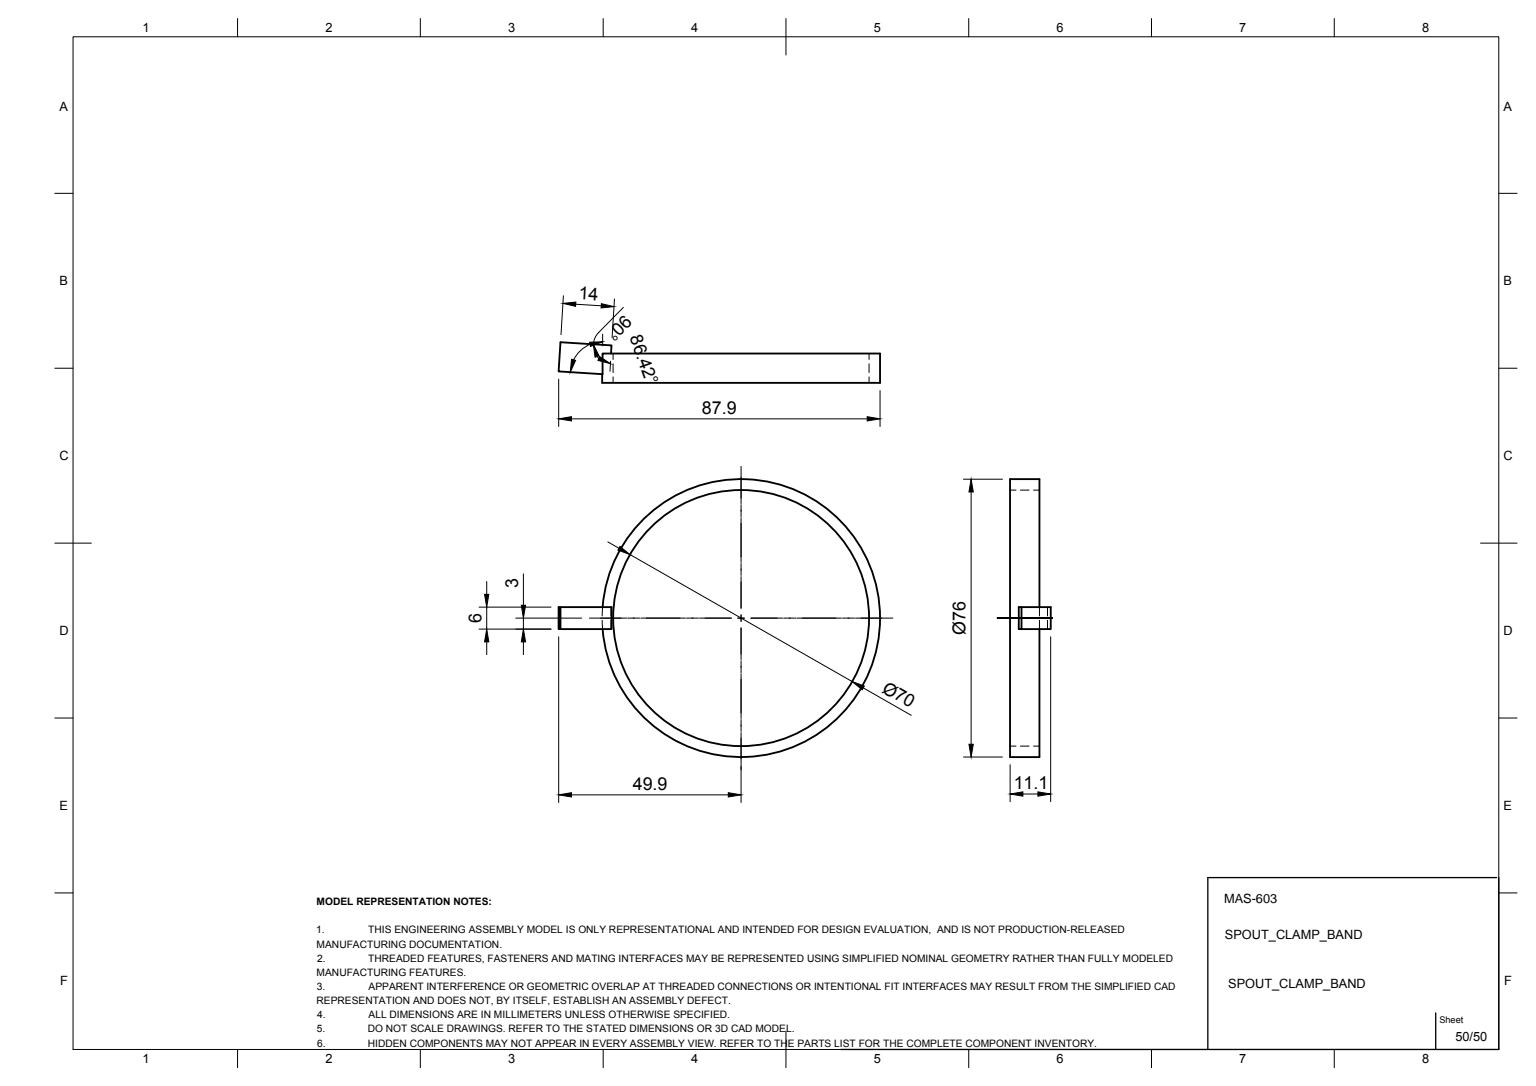
ISO-10303-21;
HEADER;
FILE_DESCRIPTION((''),'2;1');
FILE_NAME('SPOUT_CLAMP_BAND.step','2026-10-01T22:06:14-07:00',(''),(''),'','','');
FILE_SCHEMA (('AUTOMOTIVE_DESIGN { 1 0 10303 214 3 1 1 }'));
ENDSEC;
DATA;
#10=MECHANICAL_DESIGN_GEOMETRIC_PRESENTATION_REPRESENTATION('',(#1029),#50440);
#675=ELLIPSE('',#32186,3.80741464119683,3.8) ;
#928=SHAPE_REPRESENTATION_RELATIONSHIP('SRR','None',#50662,#973) ;
#973=ADVANCED_BREP_SHAPE_REPRESENTATION('',(#1082),#50431) ;
#1029=STYLED_ITEM('',(#50889),#1082) ;
#1082=MANIFOLD_SOLID_BREP('SPOUT_CLAMP_BAND',#28707) ;
#1398=FACE_BOUND('',#5656,.T.) ;
#1399=FACE_BOUND('',#5660,.T.) ;
#2289=PLANE('',#32184) ;
#2290=PLANE('',#32185) ;
#2291=PLANE('',#32187) ;
#2292=PLANE('',#32188) ;
#2293=PLANE('',#32189) ;
#2294=PLANE('',#32190) ;
#2295=PLANE('',#32191) ;
#2296=PLANE('',#32199) ;
#3809=FACE_OUTER_BOUND('',#5649,.T.) ;
#3810=FACE_OUTER_BOUND('',#5650,.T.) ;
#3811=FACE_OUTER_BOUND('',#5651,.T.) ;
#3812=FACE_OUTER_BOUND('',#5652,.T.) ;
#3813=FACE_OUTER_BOUND('',#5653,.T.) ;
#3814=FACE_OUTER_BOUND('',#5654,.T.) ;
#3815=FACE_OUTER_BOUND('',#5655,.T.) ;
#3816=FACE_OUTER_BOUND('',#5657,.T.) ;
#3817=FACE_OUTER_BOUND('',#5658,.T.) ;
#3818=FACE_OUTER_BOUND('',#5659,.T.) ;
#5649=EDGE_LOOP('',(#26259,#26260,#26261,#26262,#26263,#26264)) ;
#5650=EDGE_LOOP('',(#26265,#26266,#26267,#26268)) ;
#5651=EDGE_LOOP('',(#26269,#26270,#26271,#26272)) ;
#5652=EDGE_LOOP('',(#26273,#26274,#26275,#26276)) ;
#5653=EDGE_LOOP('',(#26277,#26278,#26279,#26280)) ;
#5654=EDGE_LOOP('',(#26281,#26282,#26283,#26284,#26285,#26286)) ;
#5655=EDGE_LOOP('',(#26287,#26288,#26289,#26290,#26291)) ;
#5656=EDGE_LOOP('',(#26292)) ;
#5657=EDGE_LOOP('',(#26293,#26294,#26295,#26296)) ;
#5658=EDGE_LOOP('',(#26297,#26298,#26299,#26300,#26301,#26302,#26303,#26304)) ;
#5659=EDGE_LOOP('',(#26305)) ;
#5660=EDGE_LOOP('',(#26306)) ;
#8105=LINE('',#49845,#10577) ;
#8106=LINE('',#49847,#10578) ;
#8107=LINE('',#49849,#10579) ;
#8108=LINE('',#49851,#10580) ;
#8109=LINE('',#49853,#10581) ;
#8110=LINE('',#49854,#10582) ;
#8111=LINE('',#49859,#10583) ;
#8112=LINE('',#49860,#10584) ;
#8113=LINE('',#49863,#10585) ;
#8114=LINE('',#49864,#10586) ;
#8115=LINE('',#49867,#10587) ;
#8116=LINE('',#49869,#10588) ;
#8117=LINE('',#49870,#10589) ;
#8118=LINE('',#49872,#10590) ;
#8119=LINE('',#49875,#10591) ;
#8120=LINE('',#49876,#10592) ;
#8121=LINE('',#49885,#10593) ;
#8122=LINE('',#49890,#10594) ;
#10577=VECTOR('',#40700,1.) ;
#10578=VECTOR('',#40701,1.) ;
#10579=VECTOR('',#40702,1.) ;
#10580=VECTOR('',#40703,1.) ;
#10581=VECTOR('',#40704,1.) ;
#10582=VECTOR('',#40705,1.) ;
#10583=VECTOR('',#40710,1.) ;
#10584=VECTOR('',#40711,1.) ;
#10585=VECTOR('',#40714,1.) ;
#10586=VECTOR('',#40715,1.) ;
#10587=VECTOR('',#40718,1.) ;
#10588=VECTOR('',#40719,1.) ;
#10589=VECTOR('',#40720,1.) ;
#10590=VECTOR('',#40723,1.) ;
#10591=VECTOR('',#40726,1.) ;
#10592=VECTOR('',#40727,1.) ;
#10593=VECTOR('',#40738,3.5) ;
#10594=VECTOR('',#40745,3.8) ;
#11797=CIRCLE('',#32192,3.8) ;
#11798=CIRCLE('',#32193,3.8) ;
#11799=CIRCLE('',#32194,3.5) ;
#11800=CIRCLE('',#32196,3.5) ;
#11801=CIRCLE('',#32198,3.8) ;
#14432=VERTEX_POINT('',#49843) ;
#14433=VERTEX_POINT('',#49844) ;
#14434=VERTEX_POINT('',#49846) ;
#14435=VERTEX_POINT('',#49848) ;
#14436=VERTEX_POINT('',#49850) ;
#14437=VERTEX_POINT('',#49852) ;
#14438=VERTEX_POINT('',#49856) ;
#14439=VERTEX_POINT('',#49858) ;
#14440=VERTEX_POINT('',#49862) ;
#14441=VERTEX_POINT('',#49866) ;
#14442=VERTEX_POINT('',#49868) ;
#14443=VERTEX_POINT('',#49874) ;
#14444=VERTEX_POINT('',#49878) ;
#14445=VERTEX_POINT('',#49881) ;
#14446=VERTEX_POINT('',#49884) ;
#14447=VERTEX_POINT('',#49888) ;
#18395=EDGE_CURVE('',#14432,#14433,#8105,.T.) ;
#18396=EDGE_CURVE('',#14434,#14432,#8106,.T.) ;
#18397=EDGE_CURVE('',#14435,#14434,#8107,.T.) ;
#18398=EDGE_CURVE('',#14436,#14435,#8108,.T.) ;
#18399=EDGE_CURVE('',#14436,#14437,#8109,.T.) ;
#18400=EDGE_CURVE('',#14433,#14437,#8110,.T.) ;
#18401=EDGE_CURVE('',#14438,#14434,#675,.T.) ;
#18402=EDGE_CURVE('',#14439,#14438,#8111,.T.) ;
#18403=EDGE_CURVE('',#14435,#14439,#8112,.T.) ;
#18404=EDGE_CURVE('',#14439,#14440,#8113,.T.) ;
#18405=EDGE_CURVE('',#14440,#14436,#8114,.T.) ;
#18406=EDGE_CURVE('',#14433,#14441,#8115,.T.) ;
#18407=EDGE_CURVE('',#14437,#14442,#8116,.T.) ;
#18408=EDGE_CURVE('',#14442,#14441,#8117,.T.) ;
#18409=EDGE_CURVE('',#14440,#14442,#8118,.T.) ;
#18410=EDGE_CURVE('',#14441,#14443,#8119,.T.) ;
#18411=EDGE_CURVE('',#14443,#14438,#8120,.T.) ;
#18412=EDGE_CURVE('',#14443,#14444,#11797,.T.) ;
#18413=EDGE_CURVE('',#14444,#14432,#11798,.T.) ;
#18414=EDGE_CURVE('',#14445,#14445,#11799,.T.) ;
#18415=EDGE_CURVE('',#14445,#14446,#8121,.T.) ;
#18416=EDGE_CURVE('',#14446,#14446,#11800,.T.) ;
#18417=EDGE_CURVE('',#14447,#14447,#11801,.T.) ;
#18418=EDGE_CURVE('',#14447,#14444,#8122,.T.) ;
#26259=ORIENTED_EDGE('',*,*,#18395,.F.) ;
#26260=ORIENTED_EDGE('',*,*,#18396,.F.) ;
#26261=ORIENTED_EDGE('',*,*,#18397,.F.) ;
#26262=ORIENTED_EDGE('',*,*,#18398,.F.) ;
#26263=ORIENTED_EDGE('',*,*,#18399,.T.) ;
#26264=ORIENTED_EDGE('',*,*,#18400,.F.) ;
#26265=ORIENTED_EDGE('',*,*,#18401,.F.) ;
#26266=ORIENTED_EDGE('',*,*,#18402,.F.) ;
#26267=ORIENTED_EDGE('',*,*,#18403,.F.) ;
#26268=ORIENTED_EDGE('',*,*,#18397,.T.) ;
#26269=ORIENTED_EDGE('',*,*,#18403,.T.) ;
#26270=ORIENTED_EDGE('',*,*,#18404,.T.) ;
#26271=ORIENTED_EDGE('',*,*,#18405,.T.) ;
#26272=ORIENTED_EDGE('',*,*,#18398,.T.) ;
#26273=ORIENTED_EDGE('',*,*,#18406,.F.) ;
#26274=ORIENTED_EDGE('',*,*,#18400,.T.) ;
#26275=ORIENTED_EDGE('',*,*,#18407,.T.) ;
#26276=ORIENTED_EDGE('',*,*,#18408,.T.) ;
#26277=ORIENTED_EDGE('',*,*,#18409,.T.) ;
#26278=ORIENTED_EDGE('',*,*,#18407,.F.) ;
#26279=ORIENTED_EDGE('',*,*,#18399,.F.) ;
#26280=ORIENTED_EDGE('',*,*,#18405,.F.) ;
#26281=ORIENTED_EDGE('',*,*,#18410,.F.) ;
#26282=ORIENTED_EDGE('',*,*,#18408,.F.) ;
#26283=ORIENTED_EDGE('',*,*,#18409,.F.) ;
#26284=ORIENTED_EDGE('',*,*,#18404,.F.) ;
#26285=ORIENTED_EDGE('',*,*,#18402,.T.) ;
#26286=ORIENTED_EDGE('',*,*,#18411,.F.) ;
#26287=ORIENTED_EDGE('',*,*,#18395,.T.) ;
#26288=ORIENTED_EDGE('',*,*,#18406,.T.) ;
#26289=ORIENTED_EDGE('',*,*,#18410,.T.) ;
#26290=ORIENTED_EDGE('',*,*,#18412,.T.) ;
#26291=ORIENTED_EDGE('',*,*,#18413,.T.) ;
#26292=ORIENTED_EDGE('',*,*,#18414,.T.) ;
#26293=ORIENTED_EDGE('',*,*,#18414,.F.) ;
#26294=ORIENTED_EDGE('',*,*,#18415,.T.) ;
#26295=ORIENTED_EDGE('',*,*,#18416,.F.) ;
#26296=ORIENTED_EDGE('',*,*,#18415,.F.) ;
#26297=ORIENTED_EDGE('',*,*,#18417,.F.) ;
#26298=ORIENTED_EDGE('',*,*,#18418,.T.) ;
#26299=ORIENTED_EDGE('',*,*,#18412,.F.) ;
#26300=ORIENTED_EDGE('',*,*,#18411,.T.) ;
#26301=ORIENTED_EDGE('',*,*,#18401,.T.) ;
#26302=ORIENTED_EDGE('',*,*,#18396,.T.) ;
#26303=ORIENTED_EDGE('',*,*,#18413,.F.) ;
#26304=ORIENTED_EDGE('',*,*,#18418,.F.) ;
#26305=ORIENTED_EDGE('',*,*,#18417,.T.) ;
#26306=ORIENTED_EDGE('',*,*,#18416,.T.) ;
#27052=CYLINDRICAL_SURFACE('',#32195,3.5) ;
#27053=CYLINDRICAL_SURFACE('',#32197,3.8) ;
#28544=ADVANCED_FACE('',(#3809),#2289,.F.) ;
#28545=ADVANCED_FACE('',(#3810),#2290,.F.) ;
#28546=ADVANCED_FACE('',(#3811),#2291,.T.) ;
#28547=ADVANCED_FACE('',(#3812),#2292,.F.) ;
#28548=ADVANCED_FACE('',(#3813),#2293,.F.) ;
#28549=ADVANCED_FACE('',(#3814),#2294,.F.) ;
#28550=ADVANCED_FACE('',(#3815,#1398),#2295,.T.) ;
#28551=ADVANCED_FACE('',(#3816),#27052,.F.) ;
#28552=ADVANCED_FACE('',(#3817),#27053,.T.) ;
#28553=ADVANCED_FACE('',(#3818,#1399),#2296,.T.) ;
#28707=CLOSED_SHELL('',(#28544,#28545,#28546,#28547,#28548,#28549,#28550,
#28551,#28552,#28553)) ;
#32183=AXIS2_PLACEMENT_3D('',#49841,#40696,#40697) ;
#32184=AXIS2_PLACEMENT_3D('',#49842,#40698,#40699) ;
#32185=AXIS2_PLACEMENT_3D('',#49855,#40706,#40707) ;
#32186=AXIS2_PLACEMENT_3D('',#49857,#40708,#40709) ;
#32187=AXIS2_PLACEMENT_3D('',#49861,#40712,#40713) ;
#32188=AXIS2_PLACEMENT_3D('',#49865,#40716,#40717) ;
#32189=AXIS2_PLACEMENT_3D('',#49871,#40721,#40722) ;
#32190=AXIS2_PLACEMENT_3D('',#49873,#40724,#40725) ;
#32191=AXIS2_PLACEMENT_3D('',#49877,#40728,#40729) ;
#32192=AXIS2_PLACEMENT_3D('',#49879,#40730,#40731) ;
#32193=AXIS2_PLACEMENT_3D('',#49880,#40732,#40733) ;
#32194=AXIS2_PLACEMENT_3D('',#49882,#40734,#40735) ;
#32195=AXIS2_PLACEMENT_3D('',#49883,#40736,#40737) ;
#32196=AXIS2_PLACEMENT_3D('',#49886,#40739,#40740) ;
#32197=AXIS2_PLACEMENT_3D('',#49887,#40741,#40742) ;
#32198=AXIS2_PLACEMENT_3D('',#49889,#40743,#40744) ;
#32199=AXIS2_PLACEMENT_3D('',#49891,#40746,#40747) ;
#40696=DIRECTION('axis',(0.,0.,1.)) ;
#40697=DIRECTION('refdir',(1.,0.,0.)) ;
#40698=DIRECTION('center_axis',(0.,1.,0.)) ;
#40699=DIRECTION('ref_axis',(0.,0.,1.)) ;
#40700=DIRECTION('',(-0.0623782861551789,0.,-0.998052578482889)) ;
#40701=DIRECTION('',(-0.998052578482889,0.,0.0623782861551789)) ;
#40702=DIRECTION('',(0.,0.,-1.)) ;
#40703=DIRECTION('',(1.,0.,0.)) ;
#40704=DIRECTION('',(0.,0.,-1.)) ;
#40705=DIRECTION('',(-1.,0.,0.)) ;
#40706=DIRECTION('center_axis',(-1.,0.,0.)) ;
#40707=DIRECTION('ref_axis',(0.,0.,1.)) ;
#40708=DIRECTION('center_axis',(1.,0.,0.)) ;
#40709=DIRECTION('ref_axis',(0.,0.,1.)) ;
#40710=DIRECTION('',(0.,0.,-1.)) ;
#40711=DIRECTION('',(0.,1.,0.)) ;
#40712=DIRECTION('center_axis',(0.,0.,1.)) ;
#40713=DIRECTION('ref_axis',(1.,0.,0.)) ;
#40714=DIRECTION('',(-1.,0.,0.)) ;
#40715=DIRECTION('',(0.,-1.,0.)) ;
#40716=DIRECTION('center_axis',(0.,0.,1.)) ;
#40717=DIRECTION('ref_axis',(1.,0.,0.)) ;
#40718=DIRECTION('',(0.,1.,0.)) ;
#40719=DIRECTION('',(0.,1.,0.)) ;
#40720=DIRECTION('',(1.,0.,0.)) ;
#40721=DIRECTION('center_axis',(1.,0.,0.)) ;
#40722=DIRECTION('ref_axis',(0.,0.,-1.)) ;
#40723=DIRECTION('',(0.,0.,-1.)) ;
#40724=DIRECTION('center_axis',(0.,-1.,0.)) ;
#40725=DIRECTION('ref_axis',(0.,0.,-1.)) ;
#40726=DIRECTION('',(0.0623782861551789,0.,0.998052578482889)) ;
#40727=DIRECTION('',(0.998052578482889,0.,-0.0623782861551789)) ;
#40728=DIRECTION('center_axis',(-0.998052578482889,0.,0.0623782861551789)) ;
#40729=DIRECTION('ref_axis',(-0.0623782861551789,0.,-0.998052578482889)) ;
#40730=DIRECTION('center_axis',(-0.998052578482889,0.,0.0623782861551789)) ;
#40731=DIRECTION('ref_axis',(0.0623782861551789,0.,0.998052578482889)) ;
#40732=DIRECTION('center_axis',(-0.998052578482889,0.,0.0623782861551789)) ;
#40733=DIRECTION('ref_axis',(0.0623782861551789,0.,0.998052578482889)) ;
#40734=DIRECTION('center_axis',(0.998052578482889,0.,-0.0623782861551789)) ;
#40735=DIRECTION('ref_axis',(0.0623782861551792,0.,0.998052578482889)) ;
#40736=DIRECTION('center_axis',(0.998052578482889,0.,-0.0623782861551792)) ;
#40737=DIRECTION('ref_axis',(0.0623782861551792,0.,0.998052578482889)) ;
#40738=DIRECTION('',(0.998052578482889,0.,-0.0623782861551792)) ;
#40739=DIRECTION('center_axis',(-0.998052578482889,0.,0.0623782861551789)) ;
#40740=DIRECTION('ref_axis',(0.0623782861551792,0.,0.998052578482889)) ;
#40741=DIRECTION('center_axis',(0.998052578482889,0.,-0.0623782861551789)) ;
#40742=DIRECTION('ref_axis',(0.0623782861551789,0.,0.998052578482889)) ;
#40743=DIRECTION('center_axis',(0.998052578482889,0.,-0.0623782861551789)) ;
#40744=DIRECTION('ref_axis',(0.0623782861551789,0.,0.998052578482889)) ;
#40745=DIRECTION('',(-0.998052578482889,0.,0.0623782861551789)) ;
#40746=DIRECTION('center_axis',(0.998052578482889,0.,-0.0623782861551789)) ;
#40747=DIRECTION('ref_axis',(0.0623782861551789,0.,0.998052578482889)) ;
#49841=CARTESIAN_POINT('',(0.,0.,0.)) ;
#49842=CARTESIAN_POINT('Origin',(60.4,-0.3,15.5)) ;
#49843=CARTESIAN_POINT('',(60.2362976425517,-0.3,15.030762280827)) ;
#49844=CARTESIAN_POINT('',(60.221875,-0.3,14.8)) ;
#49845=CARTESIAN_POINT('',(60.1330739299611,-0.3,13.3791828793774)) ;
#49846=CARTESIAN_POINT('',(60.8,-0.3,14.9955308834865)) ;
#49847=CARTESIAN_POINT('',(60.6362976425517,-0.3,15.005762280827)) ;
#49848=CARTESIAN_POINT('',(60.8,-0.3,16.2)) ;
#49849=CARTESIAN_POINT('',(60.8,-0.3,15.5)) ;
#49850=CARTESIAN_POINT('',(60.,-0.3,16.2)) ;
#49851=CARTESIAN_POINT('',(60.4,-0.3,16.2)) ;
#49852=CARTESIAN_POINT('',(60.,-0.3,14.8)) ;
#49853=CARTESIAN_POINT('',(60.,-0.3,15.5)) ;
#49854=CARTESIAN_POINT('',(60.4,-0.3,14.8)) ;
#49855=CARTESIAN_POINT('Origin',(60.8,0.,15.5)) ;
#49856=CARTESIAN_POINT('',(60.8,0.3,14.9955308834865)) ;
#49857=CARTESIAN_POINT('Origin',(60.8,0.,11.2)) ;
#49858=CARTESIAN_POINT('',(60.8,0.3,16.2)) ;
#49859=CARTESIAN_POINT('',(60.8,0.3,15.5)) ;
#49860=CARTESIAN_POINT('',(60.8,0.,16.2)) ;
#49861=CARTESIAN_POINT('Origin',(60.4,0.,16.2)) ;
#49862=CARTESIAN_POINT('',(60.,0.3,16.2)) ;
#49863=CARTESIAN_POINT('',(60.4,0.3,16.2)) ;
#49864=CARTESIAN_POINT('',(60.,0.,16.2)) ;
#49865=CARTESIAN_POINT('Origin',(60.4,0.,14.8)) ;
#49866=CARTESIAN_POINT('',(60.221875,0.3,14.8)) ;
#49867=CARTESIAN_POINT('',(60.221875,0.,14.8)) ;
#49868=CARTESIAN_POINT('',(60.,0.3,14.8)) ;
#49869=CARTESIAN_POINT('',(60.,0.,14.8)) ;
#49870=CARTESIAN_POINT('',(60.4,0.3,14.8)) ;
#49871=CARTESIAN_POINT('Origin',(60.,0.,15.5)) ;
#49872=CARTESIAN_POINT('',(60.,0.3,15.5)) ;
#49873=CARTESIAN_POINT('Origin',(60.4,0.3,15.5)) ;
#49874=CARTESIAN_POINT('',(60.2362976425517,0.3,15.030762280827)) ;
#49875=CARTESIAN_POINT('',(60.1330739299611,0.3,13.3791828793774)) ;
#49876=CARTESIAN_POINT('',(60.6362976425517,0.3,15.005762280827)) ;
#49877=CARTESIAN_POINT('Origin',(60.,0.,11.25)) ;
#49878=CARTESIAN_POINT('',(59.7629625126103,4.65365783675994E-16,7.45740020176502)) ;
#49879=CARTESIAN_POINT('Origin',(60.,0.,11.25)) ;
#49880=CARTESIAN_POINT('Origin',(60.,0.,11.25)) ;
#49881=CARTESIAN_POINT('',(59.7816759984569,4.28626379701574E-16,7.75681597530989)) ;
#49882=CARTESIAN_POINT('Origin',(60.,0.,11.25)) ;
#49883=CARTESIAN_POINT('Origin',(60.4,0.,11.225)) ;
#49884=CARTESIAN_POINT('',(60.5816759984569,-4.28626379701574E-16,7.70681597530989)) ;
#49885=CARTESIAN_POINT('',(60.1816759984569,4.28626379701574E-16,7.73181597530989)) ;
#49886=CARTESIAN_POINT('Origin',(60.8,0.,11.2)) ;
#49887=CARTESIAN_POINT('Origin',(60.4,0.,11.225)) ;
#49888=CARTESIAN_POINT('',(60.5629625126103,4.65365783675994E-16,7.40740020176502)) ;
#49889=CARTESIAN_POINT('Origin',(60.8,0.,11.2)) ;
#49890=CARTESIAN_POINT('',(60.1629625126103,4.65365783675994E-16,7.43240020176502)) ;
#49891=CARTESIAN_POINT('Origin',(60.8,0.,11.2)) ;
#50378=UNCERTAINTY_MEASURE_WITH_UNIT(LENGTH_MEASURE(0.001),#50441,
'DISTANCE_ACCURACY_VALUE',
'Maximum model space distance between geometric entities at asserted c
onnectivities') ;
#50387=UNCERTAINTY_MEASURE_WITH_UNIT(LENGTH_MEASURE(0.001),#50441,
'DISTANCE_ACCURACY_VALUE',
'Maximum model space distance between geometric entities at asserted c
onnectivities') ;
#50431=(
GEOMETRIC_REPRESENTATION_CONTEXT(3)
GLOBAL_UNCERTAINTY_ASSIGNED_CONTEXT((#50378))
GLOBAL_UNIT_ASSIGNED_CONTEXT((#50441,#50443,#50444))
REPRESENTATION_CONTEXT('','3D')
) ;
#50440=(
GEOMETRIC_REPRESENTATION_CONTEXT(3)
GLOBAL_UNCERTAINTY_ASSIGNED_CONTEXT((#50387))
GLOBAL_UNIT_ASSIGNED_CONTEXT((#50441,#50443,#50444))
REPRESENTATION_CONTEXT('','3D')
) ;
#50441=(
LENGTH_UNIT()
NAMED_UNIT(*)
SI_UNIT(.CENTI.,.METRE.)
) ;
#50443=(
NAMED_UNIT(*)
PLANE_ANGLE_UNIT()
SI_UNIT($,.RADIAN.)
) ;
#50444=(
NAMED_UNIT(*)
SI_UNIT($,.STERADIAN.)
SOLID_ANGLE_UNIT()
) ;
#50488=SHAPE_DEFINITION_REPRESENTATION(#50578,#50662) ;
#50578=PRODUCT_DEFINITION_SHAPE('',$,#50715) ;
#50662=SHAPE_REPRESENTATION('',(#32183),#50431) ;
#50671=PRODUCT_DEFINITION_CONTEXT('part definition',#50829,'design') ;
#50715=PRODUCT_DEFINITION('SPOUT_CLAMP_BAND','SPOUT_CLAMP_BAND',
#50767,#50671) ;
#50767=PRODUCT_DEFINITION_FORMATION('',$,#50874) ;
#50829=APPLICATION_CONTEXT(
'Core Data for Automotive Mechanical Design Process') ;
#50830=PRODUCT_CONTEXT('part definition',#50829,'mechanical') ;
#50874=PRODUCT('SPOUT_CLAMP_BAND','SPOUT_CLAMP_BAND',$,(#50830)) ;
#50889=PRESENTATION_STYLE_ASSIGNMENT((#50896)) ;
#50896=SURFACE_STYLE_USAGE(.BOTH.,#50903) ;
#50903=SURFACE_SIDE_STYLE('',(#50910)) ;
#50910=SURFACE_STYLE_FILL_AREA(#50917) ;
#50917=FILL_AREA_STYLE('Stainless Steel - Satin',(#50924)) ;
#50924=FILL_AREA_STYLE_COLOUR('Stainless Steel - Satin',#50931) ;
#50931=COLOUR_RGB('Stainless Steel - Satin', 0.72549020, 0.75294118, 0.79215686) ;
ENDSEC;
END-ISO-10303-21;
